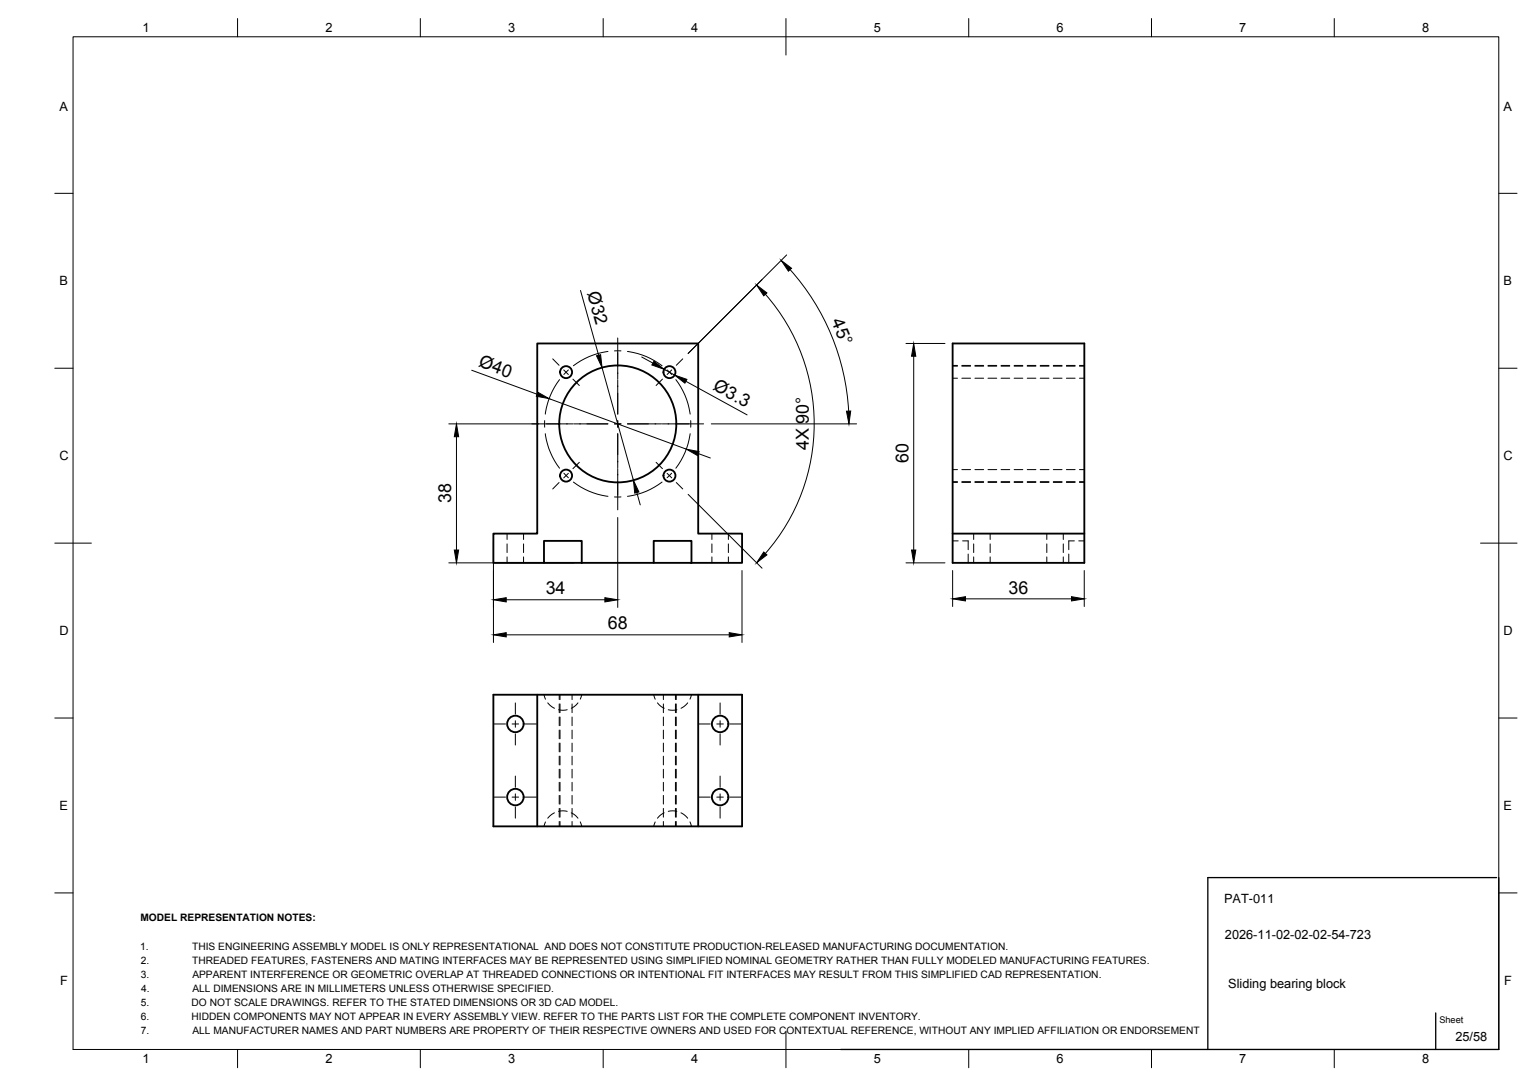
ISO-10303-21;
HEADER;
/* Generated by software containing ST-Developer
 * from STEP Tools, Inc. (www.steptools.com) 
 */

FILE_DESCRIPTION(
/* description */ ('Belt tension measurement rig'),
/* implementation_level */ '2;1');

FILE_NAME(
/* name */ 'Sliding bearing block.step',
/* time_stamp */ '2026-10-28T03:24:44-07:00',
/* author */ (''),
/* organization */ (''),
/* preprocessor_version */ 'ST-DEVELOPER v20.2',
/* originating_system */ 'Autodesk Translation Framework v15.17.0.0',
/* authorisation */ '');

FILE_SCHEMA (('AUTOMOTIVE_DESIGN { 1 0 10303 214 3 1 1 }'));
ENDSEC;

DATA;
#10=MECHANICAL_DESIGN_GEOMETRIC_PRESENTATION_REPRESENTATION('',(#720),#23587);
#602=SHAPE_REPRESENTATION_RELATIONSHIP('SRR','None',#23849,#657);
#657=ADVANCED_BREP_SHAPE_REPRESENTATION('',(#790),#23547);
#720=STYLED_ITEM('',(#24211),#790);
#790=MANIFOLD_SOLID_BREP('Body1',#12225);
#936=FACE_BOUND('',#2421,.T.);
#937=FACE_BOUND('',#2422,.T.);
#938=FACE_BOUND('',#2423,.T.);
#939=FACE_BOUND('',#2424,.T.);
#940=FACE_BOUND('',#2425,.T.);
#941=FACE_BOUND('',#2427,.T.);
#942=FACE_BOUND('',#2428,.T.);
#943=FACE_BOUND('',#2429,.T.);
#944=FACE_BOUND('',#2430,.T.);
#945=FACE_BOUND('',#2431,.T.);
#946=FACE_BOUND('',#2437,.T.);
#947=FACE_BOUND('',#2438,.T.);
#948=FACE_BOUND('',#2440,.T.);
#949=FACE_BOUND('',#2441,.T.);
#950=FACE_BOUND('',#2448,.T.);
#951=FACE_BOUND('',#2449,.T.);
#952=FACE_BOUND('',#2450,.T.);
#953=FACE_BOUND('',#2451,.T.);
#1161=PLANE('',#13409);
#1162=PLANE('',#13413);
#1163=PLANE('',#13417);
#1164=PLANE('',#13421);
#1165=PLANE('',#13425);
#1166=PLANE('',#13426);
#1167=PLANE('',#13439);
#1168=PLANE('',#13440);
#1169=PLANE('',#13441);
#1170=PLANE('',#13442);
#1171=PLANE('',#13443);
#1172=PLANE('',#13444);
#1173=PLANE('',#13445);
#1174=PLANE('',#13446);
#1596=FACE_OUTER_BOUND('',#2407,.T.);
#1597=FACE_OUTER_BOUND('',#2408,.T.);
#1598=FACE_OUTER_BOUND('',#2409,.T.);
#1599=FACE_OUTER_BOUND('',#2410,.T.);
#1600=FACE_OUTER_BOUND('',#2411,.T.);
#1601=FACE_OUTER_BOUND('',#2412,.T.);
#1602=FACE_OUTER_BOUND('',#2413,.T.);
#1603=FACE_OUTER_BOUND('',#2414,.T.);
#1604=FACE_OUTER_BOUND('',#2415,.T.);
#1605=FACE_OUTER_BOUND('',#2416,.T.);
#1606=FACE_OUTER_BOUND('',#2417,.T.);
#1607=FACE_OUTER_BOUND('',#2418,.T.);
#1608=FACE_OUTER_BOUND('',#2419,.T.);
#1609=FACE_OUTER_BOUND('',#2420,.T.);
#1610=FACE_OUTER_BOUND('',#2426,.T.);
#1611=FACE_OUTER_BOUND('',#2432,.T.);
#1612=FACE_OUTER_BOUND('',#2433,.T.);
#1613=FACE_OUTER_BOUND('',#2434,.T.);
#1614=FACE_OUTER_BOUND('',#2435,.T.);
#1615=FACE_OUTER_BOUND('',#2436,.T.);
#1616=FACE_OUTER_BOUND('',#2439,.T.);
#1617=FACE_OUTER_BOUND('',#2442,.T.);
#1618=FACE_OUTER_BOUND('',#2443,.T.);
#1619=FACE_OUTER_BOUND('',#2444,.T.);
#1620=FACE_OUTER_BOUND('',#2445,.T.);
#1621=FACE_OUTER_BOUND('',#2446,.T.);
#1622=FACE_OUTER_BOUND('',#2447,.T.);
#2407=EDGE_LOOP('',(#8980,#8981,#8982,#8983));
#2408=EDGE_LOOP('',(#8984,#8985,#8986,#8987));
#2409=EDGE_LOOP('',(#8988,#8989,#8990,#8991));
#2410=EDGE_LOOP('',(#8992,#8993,#8994,#8995));
#2411=EDGE_LOOP('',(#8996,#8997,#8998,#8999));
#2412=EDGE_LOOP('',(#9000,#9001));
#2413=EDGE_LOOP('',(#9002,#9003,#9004,#9005));
#2414=EDGE_LOOP('',(#9006,#9007));
#2415=EDGE_LOOP('',(#9008,#9009,#9010,#9011));
#2416=EDGE_LOOP('',(#9012,#9013));
#2417=EDGE_LOOP('',(#9014,#9015,#9016,#9017));
#2418=EDGE_LOOP('',(#9018,#9019));
#2419=EDGE_LOOP('',(#9020,#9021,#9022,#9023));
#2420=EDGE_LOOP('',(#9024,#9025,#9026,#9027,#9028,#9029,#9030,#9031,#9032,
#9033,#9034,#9035,#9036,#9037,#9038,#9039));
#2421=EDGE_LOOP('',(#9040));
#2422=EDGE_LOOP('',(#9041));
#2423=EDGE_LOOP('',(#9042));
#2424=EDGE_LOOP('',(#9043));
#2425=EDGE_LOOP('',(#9044));
#2426=EDGE_LOOP('',(#9045,#9046,#9047,#9048,#9049,#9050,#9051,#9052,#9053,
#9054,#9055,#9056,#9057,#9058,#9059,#9060));
#2427=EDGE_LOOP('',(#9061));
#2428=EDGE_LOOP('',(#9062));
#2429=EDGE_LOOP('',(#9063));
#2430=EDGE_LOOP('',(#9064));
#2431=EDGE_LOOP('',(#9065));
#2432=EDGE_LOOP('',(#9066,#9067,#9068,#9069));
#2433=EDGE_LOOP('',(#9070,#9071,#9072,#9073));
#2434=EDGE_LOOP('',(#9074,#9075,#9076,#9077));
#2435=EDGE_LOOP('',(#9078,#9079,#9080,#9081));
#2436=EDGE_LOOP('',(#9082,#9083,#9084,#9085));
#2437=EDGE_LOOP('',(#9086));
#2438=EDGE_LOOP('',(#9087));
#2439=EDGE_LOOP('',(#9088,#9089,#9090,#9091));
#2440=EDGE_LOOP('',(#9092));
#2441=EDGE_LOOP('',(#9093));
#2442=EDGE_LOOP('',(#9094,#9095,#9096,#9097));
#2443=EDGE_LOOP('',(#9098,#9099,#9100,#9101));
#2444=EDGE_LOOP('',(#9102,#9103,#9104,#9105));
#2445=EDGE_LOOP('',(#9106,#9107,#9108,#9109));
#2446=EDGE_LOOP('',(#9110,#9111,#9112,#9113));
#2447=EDGE_LOOP('',(#9114,#9115,#9116,#9117,#9118,#9119,#9120,#9121,#9122,
#9123,#9124,#9125));
#2448=EDGE_LOOP('',(#9126));
#2449=EDGE_LOOP('',(#9127));
#2450=EDGE_LOOP('',(#9128));
#2451=EDGE_LOOP('',(#9129));
#3223=LINE('',#20113,#3974);
#3224=LINE('',#20119,#3975);
#3225=LINE('',#20125,#3976);
#3226=LINE('',#20131,#3977);
#3227=LINE('',#20137,#3978);
#3228=LINE('',#20142,#3979);
#3229=LINE('',#20146,#3980);
#3230=LINE('',#20149,#3981);
#3231=LINE('',#20153,#3982);
#3232=LINE('',#20157,#3983);
#3233=LINE('',#20160,#3984);
#3234=LINE('',#20164,#3985);
#3235=LINE('',#20168,#3986);
#3236=LINE('',#20171,#3987);
#3237=LINE('',#20175,#3988);
#3238=LINE('',#20179,#3989);
#3239=LINE('',#20182,#3990);
#3240=LINE('',#20185,#3991);
#3241=LINE('',#20187,#3992);
#3242=LINE('',#20189,#3993);
#3243=LINE('',#20191,#3994);
#3244=LINE('',#20193,#3995);
#3245=LINE('',#20195,#3996);
#3246=LINE('',#20197,#3997);
#3247=LINE('',#20199,#3998);
#3248=LINE('',#20200,#3999);
#3249=LINE('',#20201,#4000);
#3250=LINE('',#20204,#4001);
#3251=LINE('',#20206,#4002);
#3252=LINE('',#20208,#4003);
#3253=LINE('',#20210,#4004);
#3254=LINE('',#20212,#4005);
#3255=LINE('',#20214,#4006);
#3256=LINE('',#20216,#4007);
#3257=LINE('',#20218,#4008);
#3258=LINE('',#20219,#4009);
#3259=LINE('',#20220,#4010);
#3260=LINE('',#20225,#4011);
#3261=LINE('',#20231,#4012);
#3262=LINE('',#20237,#4013);
#3263=LINE('',#20243,#4014);
#3264=LINE('',#20246,#4015);
#3265=LINE('',#20247,#4016);
#3266=LINE('',#20249,#4017);
#3267=LINE('',#20250,#4018);
#3268=LINE('',#20252,#4019);
#3269=LINE('',#20254,#4020);
#3270=LINE('',#20256,#4021);
#3271=LINE('',#20258,#4022);
#3974=VECTOR('',#15812,0.164999999999999);
#3975=VECTOR('',#15819,0.164999999999999);
#3976=VECTOR('',#15826,0.164999999999999);
#3977=VECTOR('',#15833,0.164999999999999);
#3978=VECTOR('',#15840,1.6);
#3979=VECTOR('',#15845,1.);
#3980=VECTOR('',#15850,1.);
#3981=VECTOR('',#15853,1.);
#3982=VECTOR('',#15856,1.);
#3983=VECTOR('',#15861,1.);
#3984=VECTOR('',#15864,1.);
#3985=VECTOR('',#15867,1.);
#3986=VECTOR('',#15872,1.);
#3987=VECTOR('',#15875,1.);
#3988=VECTOR('',#15878,1.);
#3989=VECTOR('',#15883,1.);
#3990=VECTOR('',#15886,1.);
#3991=VECTOR('',#15889,1.);
#3992=VECTOR('',#15890,1.);
#3993=VECTOR('',#15891,1.);
#3994=VECTOR('',#15892,1.);
#3995=VECTOR('',#15893,1.);
#3996=VECTOR('',#15894,1.);
#3997=VECTOR('',#15895,1.);
#3998=VECTOR('',#15896,1.);
#3999=VECTOR('',#15897,1.);
#4000=VECTOR('',#15898,1.);
#4001=VECTOR('',#15901,1.);
#4002=VECTOR('',#15902,1.);
#4003=VECTOR('',#15903,1.);
#4004=VECTOR('',#15904,1.);
#4005=VECTOR('',#15905,1.);
#4006=VECTOR('',#15906,1.);
#4007=VECTOR('',#15907,1.);
#4008=VECTOR('',#15908,1.);
#4009=VECTOR('',#15909,1.);
#4010=VECTOR('',#15910,1.);
#4011=VECTOR('',#15915,0.225);
#4012=VECTOR('',#15922,0.225);
#4013=VECTOR('',#15929,0.225);
#4014=VECTOR('',#15936,0.225);
#4015=VECTOR('',#15941,1.);
#4016=VECTOR('',#15942,1.);
#4017=VECTOR('',#15945,1.);
#4018=VECTOR('',#15946,1.);
#4019=VECTOR('',#15949,1.);
#4020=VECTOR('',#15952,1.);
#4021=VECTOR('',#15955,1.);
#4022=VECTOR('',#15958,1.);
#4714=CIRCLE('',#13395,0.164999999999999);
#4715=CIRCLE('',#13396,0.164999999999999);
#4716=CIRCLE('',#13398,0.164999999999999);
#4717=CIRCLE('',#13399,0.164999999999999);
#4718=CIRCLE('',#13401,0.164999999999999);
#4719=CIRCLE('',#13402,0.164999999999999);
#4720=CIRCLE('',#13404,0.164999999999999);
#4721=CIRCLE('',#13405,0.164999999999999);
#4722=CIRCLE('',#13407,1.6);
#4723=CIRCLE('',#13408,1.6);
#4724=CIRCLE('',#13410,0.525);
#4725=CIRCLE('',#13412,0.525);
#4726=CIRCLE('',#13414,0.525);
#4727=CIRCLE('',#13416,0.525);
#4728=CIRCLE('',#13418,0.525);
#4729=CIRCLE('',#13420,0.525);
#4730=CIRCLE('',#13422,0.525);
#4731=CIRCLE('',#13424,0.525);
#4732=CIRCLE('',#13428,0.225);
#4733=CIRCLE('',#13429,0.225);
#4734=CIRCLE('',#13431,0.225);
#4735=CIRCLE('',#13432,0.225);
#4736=CIRCLE('',#13434,0.225);
#4737=CIRCLE('',#13435,0.225);
#4738=CIRCLE('',#13437,0.225);
#4739=CIRCLE('',#13438,0.225);
#5592=VERTEX_POINT('',#20110);
#5593=VERTEX_POINT('',#20112);
#5594=VERTEX_POINT('',#20116);
#5595=VERTEX_POINT('',#20118);
#5596=VERTEX_POINT('',#20122);
#5597=VERTEX_POINT('',#20124);
#5598=VERTEX_POINT('',#20128);
#5599=VERTEX_POINT('',#20130);
#5600=VERTEX_POINT('',#20134);
#5601=VERTEX_POINT('',#20136);
#5602=VERTEX_POINT('',#20140);
#5603=VERTEX_POINT('',#20141);
#5604=VERTEX_POINT('',#20145);
#5605=VERTEX_POINT('',#20147);
#5606=VERTEX_POINT('',#20151);
#5607=VERTEX_POINT('',#20152);
#5608=VERTEX_POINT('',#20156);
#5609=VERTEX_POINT('',#20158);
#5610=VERTEX_POINT('',#20162);
#5611=VERTEX_POINT('',#20163);
#5612=VERTEX_POINT('',#20167);
#5613=VERTEX_POINT('',#20169);
#5614=VERTEX_POINT('',#20173);
#5615=VERTEX_POINT('',#20174);
#5616=VERTEX_POINT('',#20178);
#5617=VERTEX_POINT('',#20180);
#5618=VERTEX_POINT('',#20184);
#5619=VERTEX_POINT('',#20186);
#5620=VERTEX_POINT('',#20188);
#5621=VERTEX_POINT('',#20190);
#5622=VERTEX_POINT('',#20192);
#5623=VERTEX_POINT('',#20194);
#5624=VERTEX_POINT('',#20196);
#5625=VERTEX_POINT('',#20198);
#5626=VERTEX_POINT('',#20203);
#5627=VERTEX_POINT('',#20205);
#5628=VERTEX_POINT('',#20207);
#5629=VERTEX_POINT('',#20209);
#5630=VERTEX_POINT('',#20211);
#5631=VERTEX_POINT('',#20213);
#5632=VERTEX_POINT('',#20215);
#5633=VERTEX_POINT('',#20217);
#5634=VERTEX_POINT('',#20222);
#5635=VERTEX_POINT('',#20224);
#5636=VERTEX_POINT('',#20228);
#5637=VERTEX_POINT('',#20230);
#5638=VERTEX_POINT('',#20234);
#5639=VERTEX_POINT('',#20236);
#5640=VERTEX_POINT('',#20240);
#5641=VERTEX_POINT('',#20242);
#6849=EDGE_CURVE('',#5592,#5592,#4714,.T.);
#6850=EDGE_CURVE('',#5592,#5593,#3223,.T.);
#6851=EDGE_CURVE('',#5593,#5593,#4715,.T.);
#6852=EDGE_CURVE('',#5594,#5594,#4716,.T.);
#6853=EDGE_CURVE('',#5594,#5595,#3224,.T.);
#6854=EDGE_CURVE('',#5595,#5595,#4717,.T.);
#6855=EDGE_CURVE('',#5596,#5596,#4718,.T.);
#6856=EDGE_CURVE('',#5596,#5597,#3225,.T.);
#6857=EDGE_CURVE('',#5597,#5597,#4719,.T.);
#6858=EDGE_CURVE('',#5598,#5598,#4720,.T.);
#6859=EDGE_CURVE('',#5598,#5599,#3226,.T.);
#6860=EDGE_CURVE('',#5599,#5599,#4721,.T.);
#6861=EDGE_CURVE('',#5600,#5600,#4722,.T.);
#6862=EDGE_CURVE('',#5600,#5601,#3227,.T.);
#6863=EDGE_CURVE('',#5601,#5601,#4723,.T.);
#6864=EDGE_CURVE('',#5602,#5603,#3228,.T.);
#6865=EDGE_CURVE('',#5603,#5602,#4724,.T.);
#6866=EDGE_CURVE('',#5604,#5602,#3229,.T.);
#6867=EDGE_CURVE('',#5605,#5604,#4725,.T.);
#6868=EDGE_CURVE('',#5603,#5605,#3230,.T.);
#6869=EDGE_CURVE('',#5606,#5607,#3231,.T.);
#6870=EDGE_CURVE('',#5607,#5606,#4726,.T.);
#6871=EDGE_CURVE('',#5608,#5606,#3232,.T.);
#6872=EDGE_CURVE('',#5609,#5608,#4727,.T.);
#6873=EDGE_CURVE('',#5607,#5609,#3233,.T.);
#6874=EDGE_CURVE('',#5610,#5611,#3234,.T.);
#6875=EDGE_CURVE('',#5611,#5610,#4728,.T.);
#6876=EDGE_CURVE('',#5612,#5610,#3235,.T.);
#6877=EDGE_CURVE('',#5613,#5612,#4729,.T.);
#6878=EDGE_CURVE('',#5611,#5613,#3236,.T.);
#6879=EDGE_CURVE('',#5614,#5615,#3237,.T.);
#6880=EDGE_CURVE('',#5615,#5614,#4730,.T.);
#6881=EDGE_CURVE('',#5616,#5614,#3238,.T.);
#6882=EDGE_CURVE('',#5617,#5616,#4731,.T.);
#6883=EDGE_CURVE('',#5615,#5617,#3239,.T.);
#6884=EDGE_CURVE('',#5605,#5618,#3240,.T.);
#6885=EDGE_CURVE('',#5618,#5619,#3241,.T.);
#6886=EDGE_CURVE('',#5619,#5620,#3242,.T.);
#6887=EDGE_CURVE('',#5620,#5621,#3243,.T.);
#6888=EDGE_CURVE('',#5622,#5621,#3244,.T.);
#6889=EDGE_CURVE('',#5623,#5622,#3245,.T.);
#6890=EDGE_CURVE('',#5623,#5624,#3246,.T.);
#6891=EDGE_CURVE('',#5624,#5625,#3247,.T.);
#6892=EDGE_CURVE('',#5625,#5612,#3248,.T.);
#6893=EDGE_CURVE('',#5613,#5604,#3249,.T.);
#6894=EDGE_CURVE('',#5609,#5626,#3250,.T.);
#6895=EDGE_CURVE('',#5626,#5627,#3251,.T.);
#6896=EDGE_CURVE('',#5627,#5628,#3252,.T.);
#6897=EDGE_CURVE('',#5628,#5629,#3253,.T.);
#6898=EDGE_CURVE('',#5630,#5629,#3254,.T.);
#6899=EDGE_CURVE('',#5631,#5630,#3255,.T.);
#6900=EDGE_CURVE('',#5631,#5632,#3256,.T.);
#6901=EDGE_CURVE('',#5632,#5633,#3257,.T.);
#6902=EDGE_CURVE('',#5633,#5616,#3258,.T.);
#6903=EDGE_CURVE('',#5617,#5608,#3259,.T.);
#6904=EDGE_CURVE('',#5634,#5634,#4732,.T.);
#6905=EDGE_CURVE('',#5634,#5635,#3260,.T.);
#6906=EDGE_CURVE('',#5635,#5635,#4733,.T.);
#6907=EDGE_CURVE('',#5636,#5636,#4734,.T.);
#6908=EDGE_CURVE('',#5636,#5637,#3261,.T.);
#6909=EDGE_CURVE('',#5637,#5637,#4735,.T.);
#6910=EDGE_CURVE('',#5638,#5638,#4736,.T.);
#6911=EDGE_CURVE('',#5638,#5639,#3262,.T.);
#6912=EDGE_CURVE('',#5639,#5639,#4737,.T.);
#6913=EDGE_CURVE('',#5640,#5640,#4738,.T.);
#6914=EDGE_CURVE('',#5640,#5641,#3263,.T.);
#6915=EDGE_CURVE('',#5641,#5641,#4739,.T.);
#6916=EDGE_CURVE('',#5620,#5631,#3264,.T.);
#6917=EDGE_CURVE('',#5619,#5632,#3265,.T.);
#6918=EDGE_CURVE('',#5628,#5623,#3266,.T.);
#6919=EDGE_CURVE('',#5624,#5627,#3267,.T.);
#6920=EDGE_CURVE('',#5625,#5626,#3268,.T.);
#6921=EDGE_CURVE('',#5618,#5633,#3269,.T.);
#6922=EDGE_CURVE('',#5621,#5630,#3270,.T.);
#6923=EDGE_CURVE('',#5629,#5622,#3271,.T.);
#8980=ORIENTED_EDGE('',*,*,#6849,.F.);
#8981=ORIENTED_EDGE('',*,*,#6850,.T.);
#8982=ORIENTED_EDGE('',*,*,#6851,.F.);
#8983=ORIENTED_EDGE('',*,*,#6850,.F.);
#8984=ORIENTED_EDGE('',*,*,#6852,.F.);
#8985=ORIENTED_EDGE('',*,*,#6853,.T.);
#8986=ORIENTED_EDGE('',*,*,#6854,.F.);
#8987=ORIENTED_EDGE('',*,*,#6853,.F.);
#8988=ORIENTED_EDGE('',*,*,#6855,.F.);
#8989=ORIENTED_EDGE('',*,*,#6856,.T.);
#8990=ORIENTED_EDGE('',*,*,#6857,.F.);
#8991=ORIENTED_EDGE('',*,*,#6856,.F.);
#8992=ORIENTED_EDGE('',*,*,#6858,.F.);
#8993=ORIENTED_EDGE('',*,*,#6859,.T.);
#8994=ORIENTED_EDGE('',*,*,#6860,.F.);
#8995=ORIENTED_EDGE('',*,*,#6859,.F.);
#8996=ORIENTED_EDGE('',*,*,#6861,.F.);
#8997=ORIENTED_EDGE('',*,*,#6862,.T.);
#8998=ORIENTED_EDGE('',*,*,#6863,.F.);
#8999=ORIENTED_EDGE('',*,*,#6862,.F.);
#9000=ORIENTED_EDGE('',*,*,#6864,.F.);
#9001=ORIENTED_EDGE('',*,*,#6865,.F.);
#9002=ORIENTED_EDGE('',*,*,#6866,.F.);
#9003=ORIENTED_EDGE('',*,*,#6867,.F.);
#9004=ORIENTED_EDGE('',*,*,#6868,.F.);
#9005=ORIENTED_EDGE('',*,*,#6865,.T.);
#9006=ORIENTED_EDGE('',*,*,#6869,.F.);
#9007=ORIENTED_EDGE('',*,*,#6870,.F.);
#9008=ORIENTED_EDGE('',*,*,#6871,.F.);
#9009=ORIENTED_EDGE('',*,*,#6872,.F.);
#9010=ORIENTED_EDGE('',*,*,#6873,.F.);
#9011=ORIENTED_EDGE('',*,*,#6870,.T.);
#9012=ORIENTED_EDGE('',*,*,#6874,.F.);
#9013=ORIENTED_EDGE('',*,*,#6875,.F.);
#9014=ORIENTED_EDGE('',*,*,#6876,.F.);
#9015=ORIENTED_EDGE('',*,*,#6877,.F.);
#9016=ORIENTED_EDGE('',*,*,#6878,.F.);
#9017=ORIENTED_EDGE('',*,*,#6875,.T.);
#9018=ORIENTED_EDGE('',*,*,#6879,.F.);
#9019=ORIENTED_EDGE('',*,*,#6880,.F.);
#9020=ORIENTED_EDGE('',*,*,#6881,.F.);
#9021=ORIENTED_EDGE('',*,*,#6882,.F.);
#9022=ORIENTED_EDGE('',*,*,#6883,.F.);
#9023=ORIENTED_EDGE('',*,*,#6880,.T.);
#9024=ORIENTED_EDGE('',*,*,#6866,.T.);
#9025=ORIENTED_EDGE('',*,*,#6864,.T.);
#9026=ORIENTED_EDGE('',*,*,#6868,.T.);
#9027=ORIENTED_EDGE('',*,*,#6884,.T.);
#9028=ORIENTED_EDGE('',*,*,#6885,.T.);
#9029=ORIENTED_EDGE('',*,*,#6886,.T.);
#9030=ORIENTED_EDGE('',*,*,#6887,.T.);
#9031=ORIENTED_EDGE('',*,*,#6888,.F.);
#9032=ORIENTED_EDGE('',*,*,#6889,.F.);
#9033=ORIENTED_EDGE('',*,*,#6890,.T.);
#9034=ORIENTED_EDGE('',*,*,#6891,.T.);
#9035=ORIENTED_EDGE('',*,*,#6892,.T.);
#9036=ORIENTED_EDGE('',*,*,#6876,.T.);
#9037=ORIENTED_EDGE('',*,*,#6874,.T.);
#9038=ORIENTED_EDGE('',*,*,#6878,.T.);
#9039=ORIENTED_EDGE('',*,*,#6893,.T.);
#9040=ORIENTED_EDGE('',*,*,#6861,.T.);
#9041=ORIENTED_EDGE('',*,*,#6858,.T.);
#9042=ORIENTED_EDGE('',*,*,#6855,.T.);
#9043=ORIENTED_EDGE('',*,*,#6852,.T.);
#9044=ORIENTED_EDGE('',*,*,#6849,.T.);
#9045=ORIENTED_EDGE('',*,*,#6871,.T.);
#9046=ORIENTED_EDGE('',*,*,#6869,.T.);
#9047=ORIENTED_EDGE('',*,*,#6873,.T.);
#9048=ORIENTED_EDGE('',*,*,#6894,.T.);
#9049=ORIENTED_EDGE('',*,*,#6895,.T.);
#9050=ORIENTED_EDGE('',*,*,#6896,.T.);
#9051=ORIENTED_EDGE('',*,*,#6897,.T.);
#9052=ORIENTED_EDGE('',*,*,#6898,.F.);
#9053=ORIENTED_EDGE('',*,*,#6899,.F.);
#9054=ORIENTED_EDGE('',*,*,#6900,.T.);
#9055=ORIENTED_EDGE('',*,*,#6901,.T.);
#9056=ORIENTED_EDGE('',*,*,#6902,.T.);
#9057=ORIENTED_EDGE('',*,*,#6881,.T.);
#9058=ORIENTED_EDGE('',*,*,#6879,.T.);
#9059=ORIENTED_EDGE('',*,*,#6883,.T.);
#9060=ORIENTED_EDGE('',*,*,#6903,.T.);
#9061=ORIENTED_EDGE('',*,*,#6863,.T.);
#9062=ORIENTED_EDGE('',*,*,#6860,.T.);
#9063=ORIENTED_EDGE('',*,*,#6857,.T.);
#9064=ORIENTED_EDGE('',*,*,#6854,.T.);
#9065=ORIENTED_EDGE('',*,*,#6851,.T.);
#9066=ORIENTED_EDGE('',*,*,#6904,.F.);
#9067=ORIENTED_EDGE('',*,*,#6905,.T.);
#9068=ORIENTED_EDGE('',*,*,#6906,.F.);
#9069=ORIENTED_EDGE('',*,*,#6905,.F.);
#9070=ORIENTED_EDGE('',*,*,#6907,.F.);
#9071=ORIENTED_EDGE('',*,*,#6908,.T.);
#9072=ORIENTED_EDGE('',*,*,#6909,.F.);
#9073=ORIENTED_EDGE('',*,*,#6908,.F.);
#9074=ORIENTED_EDGE('',*,*,#6910,.F.);
#9075=ORIENTED_EDGE('',*,*,#6911,.T.);
#9076=ORIENTED_EDGE('',*,*,#6912,.F.);
#9077=ORIENTED_EDGE('',*,*,#6911,.F.);
#9078=ORIENTED_EDGE('',*,*,#6913,.F.);
#9079=ORIENTED_EDGE('',*,*,#6914,.T.);
#9080=ORIENTED_EDGE('',*,*,#6915,.F.);
#9081=ORIENTED_EDGE('',*,*,#6914,.F.);
#9082=ORIENTED_EDGE('',*,*,#6916,.F.);
#9083=ORIENTED_EDGE('',*,*,#6886,.F.);
#9084=ORIENTED_EDGE('',*,*,#6917,.T.);
#9085=ORIENTED_EDGE('',*,*,#6900,.F.);
#9086=ORIENTED_EDGE('',*,*,#6906,.T.);
#9087=ORIENTED_EDGE('',*,*,#6915,.T.);
#9088=ORIENTED_EDGE('',*,*,#6918,.F.);
#9089=ORIENTED_EDGE('',*,*,#6896,.F.);
#9090=ORIENTED_EDGE('',*,*,#6919,.F.);
#9091=ORIENTED_EDGE('',*,*,#6890,.F.);
#9092=ORIENTED_EDGE('',*,*,#6909,.T.);
#9093=ORIENTED_EDGE('',*,*,#6912,.T.);
#9094=ORIENTED_EDGE('',*,*,#6891,.F.);
#9095=ORIENTED_EDGE('',*,*,#6919,.T.);
#9096=ORIENTED_EDGE('',*,*,#6895,.F.);
#9097=ORIENTED_EDGE('',*,*,#6920,.F.);
#9098=ORIENTED_EDGE('',*,*,#6885,.F.);
#9099=ORIENTED_EDGE('',*,*,#6921,.T.);
#9100=ORIENTED_EDGE('',*,*,#6901,.F.);
#9101=ORIENTED_EDGE('',*,*,#6917,.F.);
#9102=ORIENTED_EDGE('',*,*,#6916,.T.);
#9103=ORIENTED_EDGE('',*,*,#6899,.T.);
#9104=ORIENTED_EDGE('',*,*,#6922,.F.);
#9105=ORIENTED_EDGE('',*,*,#6887,.F.);
#9106=ORIENTED_EDGE('',*,*,#6918,.T.);
#9107=ORIENTED_EDGE('',*,*,#6889,.T.);
#9108=ORIENTED_EDGE('',*,*,#6923,.F.);
#9109=ORIENTED_EDGE('',*,*,#6897,.F.);
#9110=ORIENTED_EDGE('',*,*,#6923,.T.);
#9111=ORIENTED_EDGE('',*,*,#6888,.T.);
#9112=ORIENTED_EDGE('',*,*,#6922,.T.);
#9113=ORIENTED_EDGE('',*,*,#6898,.T.);
#9114=ORIENTED_EDGE('',*,*,#6867,.T.);
#9115=ORIENTED_EDGE('',*,*,#6893,.F.);
#9116=ORIENTED_EDGE('',*,*,#6877,.T.);
#9117=ORIENTED_EDGE('',*,*,#6892,.F.);
#9118=ORIENTED_EDGE('',*,*,#6920,.T.);
#9119=ORIENTED_EDGE('',*,*,#6894,.F.);
#9120=ORIENTED_EDGE('',*,*,#6872,.T.);
#9121=ORIENTED_EDGE('',*,*,#6903,.F.);
#9122=ORIENTED_EDGE('',*,*,#6882,.T.);
#9123=ORIENTED_EDGE('',*,*,#6902,.F.);
#9124=ORIENTED_EDGE('',*,*,#6921,.F.);
#9125=ORIENTED_EDGE('',*,*,#6884,.F.);
#9126=ORIENTED_EDGE('',*,*,#6904,.T.);
#9127=ORIENTED_EDGE('',*,*,#6907,.T.);
#9128=ORIENTED_EDGE('',*,*,#6910,.T.);
#9129=ORIENTED_EDGE('',*,*,#6913,.T.);
#11256=CYLINDRICAL_SURFACE('',#13394,0.164999999999999);
#11257=CYLINDRICAL_SURFACE('',#13397,0.164999999999999);
#11258=CYLINDRICAL_SURFACE('',#13400,0.164999999999999);
#11259=CYLINDRICAL_SURFACE('',#13403,0.164999999999999);
#11260=CYLINDRICAL_SURFACE('',#13406,1.6);
#11261=CYLINDRICAL_SURFACE('',#13411,0.525);
#11262=CYLINDRICAL_SURFACE('',#13415,0.525);
#11263=CYLINDRICAL_SURFACE('',#13419,0.525);
#11264=CYLINDRICAL_SURFACE('',#13423,0.525);
#11265=CYLINDRICAL_SURFACE('',#13427,0.225);
#11266=CYLINDRICAL_SURFACE('',#13430,0.225);
#11267=CYLINDRICAL_SURFACE('',#13433,0.225);
#11268=CYLINDRICAL_SURFACE('',#13436,0.225);
#11737=ADVANCED_FACE('',(#1596),#11256,.F.);
#11738=ADVANCED_FACE('',(#1597),#11257,.F.);
#11739=ADVANCED_FACE('',(#1598),#11258,.F.);
#11740=ADVANCED_FACE('',(#1599),#11259,.F.);
#11741=ADVANCED_FACE('',(#1600),#11260,.F.);
#11742=ADVANCED_FACE('',(#1601),#1161,.F.);
#11743=ADVANCED_FACE('',(#1602),#11261,.F.);
#11744=ADVANCED_FACE('',(#1603),#1162,.F.);
#11745=ADVANCED_FACE('',(#1604),#11262,.F.);
#11746=ADVANCED_FACE('',(#1605),#1163,.F.);
#11747=ADVANCED_FACE('',(#1606),#11263,.F.);
#11748=ADVANCED_FACE('',(#1607),#1164,.F.);
#11749=ADVANCED_FACE('',(#1608),#11264,.F.);
#11750=ADVANCED_FACE('',(#1609,#936,#937,#938,#939,#940),#1165,.T.);
#11751=ADVANCED_FACE('',(#1610,#941,#942,#943,#944,#945),#1166,.T.);
#11752=ADVANCED_FACE('',(#1611),#11265,.F.);
#11753=ADVANCED_FACE('',(#1612),#11266,.F.);
#11754=ADVANCED_FACE('',(#1613),#11267,.F.);
#11755=ADVANCED_FACE('',(#1614),#11268,.F.);
#11756=ADVANCED_FACE('',(#1615,#946,#947),#1167,.T.);
#11757=ADVANCED_FACE('',(#1616,#948,#949),#1168,.T.);
#11758=ADVANCED_FACE('',(#1617),#1169,.T.);
#11759=ADVANCED_FACE('',(#1618),#1170,.T.);
#11760=ADVANCED_FACE('',(#1619),#1171,.T.);
#11761=ADVANCED_FACE('',(#1620),#1172,.T.);
#11762=ADVANCED_FACE('',(#1621),#1173,.T.);
#11763=ADVANCED_FACE('',(#1622,#950,#951,#952,#953),#1174,.F.);
#12225=CLOSED_SHELL('',(#11737,#11738,#11739,#11740,#11741,#11742,#11743,
#11744,#11745,#11746,#11747,#11748,#11749,#11750,#11751,#11752,#11753,#11754,
#11755,#11756,#11757,#11758,#11759,#11760,#11761,#11762,#11763));
#13393=AXIS2_PLACEMENT_3D('',#20108,#15806,#15807);
#13394=AXIS2_PLACEMENT_3D('',#20109,#15808,#15809);
#13395=AXIS2_PLACEMENT_3D('',#20111,#15810,#15811);
#13396=AXIS2_PLACEMENT_3D('',#20114,#15813,#15814);
#13397=AXIS2_PLACEMENT_3D('',#20115,#15815,#15816);
#13398=AXIS2_PLACEMENT_3D('',#20117,#15817,#15818);
#13399=AXIS2_PLACEMENT_3D('',#20120,#15820,#15821);
#13400=AXIS2_PLACEMENT_3D('',#20121,#15822,#15823);
#13401=AXIS2_PLACEMENT_3D('',#20123,#15824,#15825);
#13402=AXIS2_PLACEMENT_3D('',#20126,#15827,#15828);
#13403=AXIS2_PLACEMENT_3D('',#20127,#15829,#15830);
#13404=AXIS2_PLACEMENT_3D('',#20129,#15831,#15832);
#13405=AXIS2_PLACEMENT_3D('',#20132,#15834,#15835);
#13406=AXIS2_PLACEMENT_3D('',#20133,#15836,#15837);
#13407=AXIS2_PLACEMENT_3D('',#20135,#15838,#15839);
#13408=AXIS2_PLACEMENT_3D('',#20138,#15841,#15842);
#13409=AXIS2_PLACEMENT_3D('',#20139,#15843,#15844);
#13410=AXIS2_PLACEMENT_3D('',#20143,#15846,#15847);
#13411=AXIS2_PLACEMENT_3D('',#20144,#15848,#15849);
#13412=AXIS2_PLACEMENT_3D('',#20148,#15851,#15852);
#13413=AXIS2_PLACEMENT_3D('',#20150,#15854,#15855);
#13414=AXIS2_PLACEMENT_3D('',#20154,#15857,#15858);
#13415=AXIS2_PLACEMENT_3D('',#20155,#15859,#15860);
#13416=AXIS2_PLACEMENT_3D('',#20159,#15862,#15863);
#13417=AXIS2_PLACEMENT_3D('',#20161,#15865,#15866);
#13418=AXIS2_PLACEMENT_3D('',#20165,#15868,#15869);
#13419=AXIS2_PLACEMENT_3D('',#20166,#15870,#15871);
#13420=AXIS2_PLACEMENT_3D('',#20170,#15873,#15874);
#13421=AXIS2_PLACEMENT_3D('',#20172,#15876,#15877);
#13422=AXIS2_PLACEMENT_3D('',#20176,#15879,#15880);
#13423=AXIS2_PLACEMENT_3D('',#20177,#15881,#15882);
#13424=AXIS2_PLACEMENT_3D('',#20181,#15884,#15885);
#13425=AXIS2_PLACEMENT_3D('',#20183,#15887,#15888);
#13426=AXIS2_PLACEMENT_3D('',#20202,#15899,#15900);
#13427=AXIS2_PLACEMENT_3D('',#20221,#15911,#15912);
#13428=AXIS2_PLACEMENT_3D('',#20223,#15913,#15914);
#13429=AXIS2_PLACEMENT_3D('',#20226,#15916,#15917);
#13430=AXIS2_PLACEMENT_3D('',#20227,#15918,#15919);
#13431=AXIS2_PLACEMENT_3D('',#20229,#15920,#15921);
#13432=AXIS2_PLACEMENT_3D('',#20232,#15923,#15924);
#13433=AXIS2_PLACEMENT_3D('',#20233,#15925,#15926);
#13434=AXIS2_PLACEMENT_3D('',#20235,#15927,#15928);
#13435=AXIS2_PLACEMENT_3D('',#20238,#15930,#15931);
#13436=AXIS2_PLACEMENT_3D('',#20239,#15932,#15933);
#13437=AXIS2_PLACEMENT_3D('',#20241,#15934,#15935);
#13438=AXIS2_PLACEMENT_3D('',#20244,#15937,#15938);
#13439=AXIS2_PLACEMENT_3D('',#20245,#15939,#15940);
#13440=AXIS2_PLACEMENT_3D('',#20248,#15943,#15944);
#13441=AXIS2_PLACEMENT_3D('',#20251,#15947,#15948);
#13442=AXIS2_PLACEMENT_3D('',#20253,#15950,#15951);
#13443=AXIS2_PLACEMENT_3D('',#20255,#15953,#15954);
#13444=AXIS2_PLACEMENT_3D('',#20257,#15956,#15957);
#13445=AXIS2_PLACEMENT_3D('',#20259,#15959,#15960);
#13446=AXIS2_PLACEMENT_3D('',#20260,#15961,#15962);
#15806=DIRECTION('axis',(0.,0.,1.));
#15807=DIRECTION('refdir',(1.,0.,0.));
#15808=DIRECTION('center_axis',(0.,1.,0.));
#15809=DIRECTION('ref_axis',(1.,0.,0.));
#15810=DIRECTION('center_axis',(0.,1.,0.));
#15811=DIRECTION('ref_axis',(1.,0.,0.));
#15812=DIRECTION('',(0.,1.,0.));
#15813=DIRECTION('center_axis',(0.,-1.,0.));
#15814=DIRECTION('ref_axis',(1.,0.,0.));
#15815=DIRECTION('center_axis',(0.,1.,0.));
#15816=DIRECTION('ref_axis',(1.,0.,0.));
#15817=DIRECTION('center_axis',(0.,1.,0.));
#15818=DIRECTION('ref_axis',(1.,0.,0.));
#15819=DIRECTION('',(0.,1.,0.));
#15820=DIRECTION('center_axis',(0.,-1.,0.));
#15821=DIRECTION('ref_axis',(1.,0.,0.));
#15822=DIRECTION('center_axis',(0.,1.,0.));
#15823=DIRECTION('ref_axis',(1.,0.,0.));
#15824=DIRECTION('center_axis',(0.,1.,0.));
#15825=DIRECTION('ref_axis',(1.,0.,0.));
#15826=DIRECTION('',(0.,1.,0.));
#15827=DIRECTION('center_axis',(0.,-1.,0.));
#15828=DIRECTION('ref_axis',(1.,0.,0.));
#15829=DIRECTION('center_axis',(0.,1.,0.));
#15830=DIRECTION('ref_axis',(1.,0.,0.));
#15831=DIRECTION('center_axis',(0.,1.,0.));
#15832=DIRECTION('ref_axis',(1.,0.,0.));
#15833=DIRECTION('',(0.,1.,0.));
#15834=DIRECTION('center_axis',(0.,-1.,0.));
#15835=DIRECTION('ref_axis',(1.,0.,0.));
#15836=DIRECTION('center_axis',(0.,1.,0.));
#15837=DIRECTION('ref_axis',(1.,0.,0.));
#15838=DIRECTION('center_axis',(0.,1.,0.));
#15839=DIRECTION('ref_axis',(1.,0.,0.));
#15840=DIRECTION('',(0.,1.,0.));
#15841=DIRECTION('center_axis',(0.,-1.,0.));
#15842=DIRECTION('ref_axis',(1.,0.,0.));
#15843=DIRECTION('center_axis',(0.,0.,1.));
#15844=DIRECTION('ref_axis',(1.,0.,0.));
#15845=DIRECTION('',(1.,0.,0.));
#15846=DIRECTION('center_axis',(0.,0.,1.));
#15847=DIRECTION('ref_axis',(1.,0.,0.));
#15848=DIRECTION('center_axis',(0.,0.,1.));
#15849=DIRECTION('ref_axis',(1.,0.,0.));
#15850=DIRECTION('',(0.,0.,1.));
#15851=DIRECTION('center_axis',(0.,0.,1.));
#15852=DIRECTION('ref_axis',(1.,0.,0.));
#15853=DIRECTION('',(0.,0.,-1.));
#15854=DIRECTION('center_axis',(0.,0.,1.));
#15855=DIRECTION('ref_axis',(1.,0.,0.));
#15856=DIRECTION('',(-1.,0.,0.));
#15857=DIRECTION('center_axis',(0.,0.,1.));
#15858=DIRECTION('ref_axis',(1.,0.,0.));
#15859=DIRECTION('center_axis',(0.,0.,1.));
#15860=DIRECTION('ref_axis',(1.,0.,0.));
#15861=DIRECTION('',(0.,0.,1.));
#15862=DIRECTION('center_axis',(0.,0.,1.));
#15863=DIRECTION('ref_axis',(1.,0.,0.));
#15864=DIRECTION('',(0.,0.,-1.));
#15865=DIRECTION('center_axis',(0.,0.,1.));
#15866=DIRECTION('ref_axis',(1.,0.,0.));
#15867=DIRECTION('',(1.,0.,0.));
#15868=DIRECTION('center_axis',(0.,0.,1.));
#15869=DIRECTION('ref_axis',(1.,0.,0.));
#15870=DIRECTION('center_axis',(0.,0.,1.));
#15871=DIRECTION('ref_axis',(1.,0.,0.));
#15872=DIRECTION('',(0.,0.,1.));
#15873=DIRECTION('center_axis',(0.,0.,1.));
#15874=DIRECTION('ref_axis',(1.,0.,0.));
#15875=DIRECTION('',(0.,0.,-1.));
#15876=DIRECTION('center_axis',(0.,0.,1.));
#15877=DIRECTION('ref_axis',(1.,0.,0.));
#15878=DIRECTION('',(-1.,0.,0.));
#15879=DIRECTION('center_axis',(0.,0.,1.));
#15880=DIRECTION('ref_axis',(1.,0.,0.));
#15881=DIRECTION('center_axis',(0.,0.,1.));
#15882=DIRECTION('ref_axis',(1.,0.,0.));
#15883=DIRECTION('',(0.,0.,1.));
#15884=DIRECTION('center_axis',(0.,0.,1.));
#15885=DIRECTION('ref_axis',(1.,0.,0.));
#15886=DIRECTION('',(0.,0.,-1.));
#15887=DIRECTION('center_axis',(0.,-1.,0.));
#15888=DIRECTION('ref_axis',(1.,0.,0.));
#15889=DIRECTION('',(1.,0.,0.));
#15890=DIRECTION('',(0.,0.,1.));
#15891=DIRECTION('',(-1.,0.,0.));
#15892=DIRECTION('',(0.,0.,1.));
#15893=DIRECTION('',(1.,0.,0.));
#15894=DIRECTION('',(0.,0.,1.));
#15895=DIRECTION('',(-1.,0.,0.));
#15896=DIRECTION('',(0.,0.,-1.));
#15897=DIRECTION('',(1.,0.,0.));
#15898=DIRECTION('',(1.,0.,0.));
#15899=DIRECTION('center_axis',(0.,1.,0.));
#15900=DIRECTION('ref_axis',(-1.,0.,0.));
#15901=DIRECTION('',(-1.,0.,0.));
#15902=DIRECTION('',(0.,0.,1.));
#15903=DIRECTION('',(1.,0.,0.));
#15904=DIRECTION('',(0.,0.,1.));
#15905=DIRECTION('',(-1.,0.,0.));
#15906=DIRECTION('',(0.,0.,1.));
#15907=DIRECTION('',(1.,0.,0.));
#15908=DIRECTION('',(0.,0.,-1.));
#15909=DIRECTION('',(-1.,0.,0.));
#15910=DIRECTION('',(-1.,0.,0.));
#15911=DIRECTION('center_axis',(0.,0.,1.));
#15912=DIRECTION('ref_axis',(1.,0.,0.));
#15913=DIRECTION('center_axis',(0.,0.,1.));
#15914=DIRECTION('ref_axis',(1.,0.,0.));
#15915=DIRECTION('',(0.,0.,1.));
#15916=DIRECTION('center_axis',(0.,0.,-1.));
#15917=DIRECTION('ref_axis',(1.,0.,0.));
#15918=DIRECTION('center_axis',(0.,0.,1.));
#15919=DIRECTION('ref_axis',(1.,0.,0.));
#15920=DIRECTION('center_axis',(0.,0.,1.));
#15921=DIRECTION('ref_axis',(1.,0.,0.));
#15922=DIRECTION('',(0.,0.,1.));
#15923=DIRECTION('center_axis',(0.,0.,-1.));
#15924=DIRECTION('ref_axis',(1.,0.,0.));
#15925=DIRECTION('center_axis',(0.,0.,1.));
#15926=DIRECTION('ref_axis',(1.,0.,0.));
#15927=DIRECTION('center_axis',(0.,0.,1.));
#15928=DIRECTION('ref_axis',(1.,0.,0.));
#15929=DIRECTION('',(0.,0.,1.));
#15930=DIRECTION('center_axis',(0.,0.,-1.));
#15931=DIRECTION('ref_axis',(1.,0.,0.));
#15932=DIRECTION('center_axis',(0.,0.,1.));
#15933=DIRECTION('ref_axis',(1.,0.,0.));
#15934=DIRECTION('center_axis',(0.,0.,1.));
#15935=DIRECTION('ref_axis',(1.,0.,0.));
#15936=DIRECTION('',(0.,0.,1.));
#15937=DIRECTION('center_axis',(0.,0.,-1.));
#15938=DIRECTION('ref_axis',(1.,0.,0.));
#15939=DIRECTION('center_axis',(0.,0.,1.));
#15940=DIRECTION('ref_axis',(1.,0.,0.));
#15941=DIRECTION('',(0.,1.,0.));
#15942=DIRECTION('',(0.,1.,0.));
#15943=DIRECTION('center_axis',(0.,0.,1.));
#15944=DIRECTION('ref_axis',(1.,0.,0.));
#15945=DIRECTION('',(0.,-1.,0.));
#15946=DIRECTION('',(0.,1.,0.));
#15947=DIRECTION('center_axis',(-1.,0.,0.));
#15948=DIRECTION('ref_axis',(0.,0.,1.));
#15949=DIRECTION('',(0.,1.,0.));
#15950=DIRECTION('center_axis',(1.,0.,0.));
#15951=DIRECTION('ref_axis',(0.,0.,-1.));
#15952=DIRECTION('',(0.,1.,0.));
#15953=DIRECTION('center_axis',(1.,0.,0.));
#15954=DIRECTION('ref_axis',(0.,1.,0.));
#15955=DIRECTION('',(0.,1.,0.));
#15956=DIRECTION('center_axis',(-1.,0.,0.));
#15957=DIRECTION('ref_axis',(0.,-1.,0.));
#15958=DIRECTION('',(0.,-1.,0.));
#15959=DIRECTION('center_axis',(0.,0.,1.));
#15960=DIRECTION('ref_axis',(1.,0.,0.));
#15961=DIRECTION('center_axis',(0.,0.,1.));
#15962=DIRECTION('ref_axis',(1.,0.,0.));
#20108=CARTESIAN_POINT('',(0.,0.,0.));
#20109=CARTESIAN_POINT('Origin',(8.5857864376269,-1.9,5.58578643762691));
#20110=CARTESIAN_POINT('',(8.42078643762691,-1.8,5.58578643762691));
#20111=CARTESIAN_POINT('Origin',(8.5857864376269,-1.8,5.58578643762691));
#20112=CARTESIAN_POINT('',(8.42078643762691,1.8,5.58578643762691));
#20113=CARTESIAN_POINT('',(8.42078643762691,-1.9,5.58578643762691));
#20114=CARTESIAN_POINT('Origin',(8.5857864376269,1.8,5.58578643762691));
#20115=CARTESIAN_POINT('Origin',(8.5857864376269,-1.9,8.4142135623731));
#20116=CARTESIAN_POINT('',(8.42078643762691,-1.8,8.4142135623731));
#20117=CARTESIAN_POINT('Origin',(8.5857864376269,-1.8,8.4142135623731));
#20118=CARTESIAN_POINT('',(8.42078643762691,1.8,8.4142135623731));
#20119=CARTESIAN_POINT('',(8.42078643762691,-1.9,8.4142135623731));
#20120=CARTESIAN_POINT('Origin',(8.5857864376269,1.8,8.4142135623731));
#20121=CARTESIAN_POINT('Origin',(11.4142135623731,-1.9,8.4142135623731));
#20122=CARTESIAN_POINT('',(11.2492135623731,-1.8,8.4142135623731));
#20123=CARTESIAN_POINT('Origin',(11.4142135623731,-1.8,8.4142135623731));
#20124=CARTESIAN_POINT('',(11.2492135623731,1.8,8.4142135623731));
#20125=CARTESIAN_POINT('',(11.2492135623731,-1.9,8.4142135623731));
#20126=CARTESIAN_POINT('Origin',(11.4142135623731,1.8,8.4142135623731));
#20127=CARTESIAN_POINT('Origin',(11.4142135623731,-1.9,5.58578643762691));
#20128=CARTESIAN_POINT('',(11.2492135623731,-1.8,5.58578643762691));
#20129=CARTESIAN_POINT('Origin',(11.4142135623731,-1.8,5.58578643762691));
#20130=CARTESIAN_POINT('',(11.2492135623731,1.8,5.58578643762691));
#20131=CARTESIAN_POINT('',(11.2492135623731,-1.9,5.58578643762691));
#20132=CARTESIAN_POINT('Origin',(11.4142135623731,1.8,5.58578643762691));
#20133=CARTESIAN_POINT('Origin',(10.,-1.9,7.));
#20134=CARTESIAN_POINT('',(8.4,-1.8,7.));
#20135=CARTESIAN_POINT('Origin',(10.,-1.8,7.));
#20136=CARTESIAN_POINT('',(8.4,1.8,7.));
#20137=CARTESIAN_POINT('',(8.4,-1.9,7.));
#20138=CARTESIAN_POINT('Origin',(10.,1.8,7.));
#20139=CARTESIAN_POINT('Origin',(11.5,-1.9,3.8));
#20140=CARTESIAN_POINT('',(10.9846117967978,-1.8,3.8));
#20141=CARTESIAN_POINT('',(12.0153882032022,-1.8,3.8));
#20142=CARTESIAN_POINT('',(9.65,-1.8,3.8));
#20143=CARTESIAN_POINT('Origin',(11.5,-1.9,3.8));
#20144=CARTESIAN_POINT('Origin',(11.5,-1.9,3.1));
#20145=CARTESIAN_POINT('',(10.9846117967978,-1.8,3.2));
#20146=CARTESIAN_POINT('',(10.9846117967978,-1.8,3.1));
#20147=CARTESIAN_POINT('',(12.0153882032022,-1.8,3.2));
#20148=CARTESIAN_POINT('Origin',(11.5,-1.9,3.2));
#20149=CARTESIAN_POINT('',(12.0153882032022,-1.8,3.1));
#20150=CARTESIAN_POINT('Origin',(8.5,1.9,3.8));
#20151=CARTESIAN_POINT('',(9.01538820320221,1.8,3.8));
#20152=CARTESIAN_POINT('',(7.98461179679779,1.8,3.8));
#20153=CARTESIAN_POINT('',(10.35,1.8,3.8));
#20154=CARTESIAN_POINT('Origin',(8.5,1.9,3.8));
#20155=CARTESIAN_POINT('Origin',(8.5,1.9,3.1));
#20156=CARTESIAN_POINT('',(9.01538820320221,1.8,3.2));
#20157=CARTESIAN_POINT('',(9.01538820320221,1.8,3.1));
#20158=CARTESIAN_POINT('',(7.98461179679779,1.8,3.2));
#20159=CARTESIAN_POINT('Origin',(8.5,1.9,3.2));
#20160=CARTESIAN_POINT('',(7.98461179679779,1.8,3.1));
#20161=CARTESIAN_POINT('Origin',(8.5,-1.9,3.8));
#20162=CARTESIAN_POINT('',(7.98461179679779,-1.8,3.8));
#20163=CARTESIAN_POINT('',(9.01538820320221,-1.8,3.8));
#20164=CARTESIAN_POINT('',(8.15,-1.8,3.8));
#20165=CARTESIAN_POINT('Origin',(8.5,-1.9,3.8));
#20166=CARTESIAN_POINT('Origin',(8.5,-1.9,3.1));
#20167=CARTESIAN_POINT('',(7.98461179679779,-1.8,3.2));
#20168=CARTESIAN_POINT('',(7.98461179679779,-1.8,3.1));
#20169=CARTESIAN_POINT('',(9.01538820320221,-1.8,3.2));
#20170=CARTESIAN_POINT('Origin',(8.5,-1.9,3.2));
#20171=CARTESIAN_POINT('',(9.01538820320221,-1.8,3.1));
#20172=CARTESIAN_POINT('Origin',(11.5,1.9,3.8));
#20173=CARTESIAN_POINT('',(12.0153882032022,1.8,3.8));
#20174=CARTESIAN_POINT('',(10.9846117967978,1.8,3.8));
#20175=CARTESIAN_POINT('',(11.85,1.8,3.8));
#20176=CARTESIAN_POINT('Origin',(11.5,1.9,3.8));
#20177=CARTESIAN_POINT('Origin',(11.5,1.9,3.1));
#20178=CARTESIAN_POINT('',(12.0153882032022,1.8,3.2));
#20179=CARTESIAN_POINT('',(12.0153882032022,1.8,3.1));
#20180=CARTESIAN_POINT('',(10.9846117967978,1.8,3.2));
#20181=CARTESIAN_POINT('Origin',(11.5,1.9,3.2));
#20182=CARTESIAN_POINT('',(10.9846117967978,1.8,3.1));
#20183=CARTESIAN_POINT('Origin',(7.8,-1.8,3.2));
#20184=CARTESIAN_POINT('',(13.4,-1.8,3.2));
#20185=CARTESIAN_POINT('',(6.6,-1.8,3.2));
#20186=CARTESIAN_POINT('',(13.4,-1.8,4.));
#20187=CARTESIAN_POINT('',(13.4,-1.8,3.2));
#20188=CARTESIAN_POINT('',(12.2,-1.8,4.));
#20189=CARTESIAN_POINT('',(13.4,-1.8,4.));
#20190=CARTESIAN_POINT('',(12.2,-1.8,9.2));
#20191=CARTESIAN_POINT('',(12.2,-1.8,3.2));
#20192=CARTESIAN_POINT('',(7.8,-1.8,9.2));
#20193=CARTESIAN_POINT('',(7.8,-1.8,9.2));
#20194=CARTESIAN_POINT('',(7.8,-1.8,4.));
#20195=CARTESIAN_POINT('',(7.8,-1.8,3.2));
#20196=CARTESIAN_POINT('',(6.6,-1.8,4.));
#20197=CARTESIAN_POINT('',(13.4,-1.8,4.));
#20198=CARTESIAN_POINT('',(6.6,-1.8,3.2));
#20199=CARTESIAN_POINT('',(6.6,-1.8,4.));
#20200=CARTESIAN_POINT('',(6.6,-1.8,3.2));
#20201=CARTESIAN_POINT('',(6.6,-1.8,3.2));
#20202=CARTESIAN_POINT('Origin',(12.2,1.8,3.2));
#20203=CARTESIAN_POINT('',(6.6,1.8,3.2));
#20204=CARTESIAN_POINT('',(6.6,1.8,3.2));
#20205=CARTESIAN_POINT('',(6.6,1.8,4.));
#20206=CARTESIAN_POINT('',(6.6,1.8,4.));
#20207=CARTESIAN_POINT('',(7.8,1.8,4.));
#20208=CARTESIAN_POINT('',(13.4,1.8,4.));
#20209=CARTESIAN_POINT('',(7.8,1.8,9.2));
#20210=CARTESIAN_POINT('',(7.8,1.8,3.2));
#20211=CARTESIAN_POINT('',(12.2,1.8,9.2));
#20212=CARTESIAN_POINT('',(12.2,1.8,9.2));
#20213=CARTESIAN_POINT('',(12.2,1.8,4.));
#20214=CARTESIAN_POINT('',(12.2,1.8,3.2));
#20215=CARTESIAN_POINT('',(13.4,1.8,4.));
#20216=CARTESIAN_POINT('',(13.4,1.8,4.));
#20217=CARTESIAN_POINT('',(13.4,1.8,3.2));
#20218=CARTESIAN_POINT('',(13.4,1.8,3.2));
#20219=CARTESIAN_POINT('',(6.6,1.8,3.2));
#20220=CARTESIAN_POINT('',(6.6,1.8,3.2));
#20221=CARTESIAN_POINT('Origin',(12.8,-1.,3.1));
#20222=CARTESIAN_POINT('',(12.575,-1.,3.2));
#20223=CARTESIAN_POINT('Origin',(12.8,-1.,3.2));
#20224=CARTESIAN_POINT('',(12.575,-1.,4.));
#20225=CARTESIAN_POINT('',(12.575,-1.,3.1));
#20226=CARTESIAN_POINT('Origin',(12.8,-1.,4.));
#20227=CARTESIAN_POINT('Origin',(7.2,1.,3.1));
#20228=CARTESIAN_POINT('',(6.975,1.,3.2));
#20229=CARTESIAN_POINT('Origin',(7.2,1.,3.2));
#20230=CARTESIAN_POINT('',(6.975,1.,4.));
#20231=CARTESIAN_POINT('',(6.975,1.,3.1));
#20232=CARTESIAN_POINT('Origin',(7.2,1.,4.));
#20233=CARTESIAN_POINT('Origin',(7.2,-1.,3.1));
#20234=CARTESIAN_POINT('',(6.975,-1.,3.2));
#20235=CARTESIAN_POINT('Origin',(7.2,-1.,3.2));
#20236=CARTESIAN_POINT('',(6.975,-1.,4.));
#20237=CARTESIAN_POINT('',(6.975,-1.,3.1));
#20238=CARTESIAN_POINT('Origin',(7.2,-1.,4.));
#20239=CARTESIAN_POINT('Origin',(12.8,1.,3.1));
#20240=CARTESIAN_POINT('',(12.575,1.,3.2));
#20241=CARTESIAN_POINT('Origin',(12.8,1.,3.2));
#20242=CARTESIAN_POINT('',(12.575,1.,4.));
#20243=CARTESIAN_POINT('',(12.575,1.,3.1));
#20244=CARTESIAN_POINT('Origin',(12.8,1.,4.));
#20245=CARTESIAN_POINT('Origin',(6.6,-1.8,4.));
#20246=CARTESIAN_POINT('',(12.2,-1.8,4.));
#20247=CARTESIAN_POINT('',(13.4,-1.8,4.));
#20248=CARTESIAN_POINT('Origin',(6.6,-1.8,4.));
#20249=CARTESIAN_POINT('',(7.8,0.,4.));
#20250=CARTESIAN_POINT('',(6.6,-1.8,4.));
#20251=CARTESIAN_POINT('Origin',(6.6,-1.8,3.2));
#20252=CARTESIAN_POINT('',(6.6,-1.8,3.2));
#20253=CARTESIAN_POINT('Origin',(13.4,-1.8,4.));
#20254=CARTESIAN_POINT('',(13.4,-1.8,3.2));
#20255=CARTESIAN_POINT('Origin',(12.2,-1.8,3.2));
#20256=CARTESIAN_POINT('',(12.2,-1.8,9.2));
#20257=CARTESIAN_POINT('Origin',(7.8,1.8,3.2));
#20258=CARTESIAN_POINT('',(7.8,1.8,9.2));
#20259=CARTESIAN_POINT('Origin',(10.,0.,9.2));
#20260=CARTESIAN_POINT('Origin',(10.,0.,3.2));
#23482=UNCERTAINTY_MEASURE_WITH_UNIT(LENGTH_MEASURE(0.001),#23588,
'DISTANCE_ACCURACY_VALUE',
'Maximum model space distance between geometric entities at asserted c
onnectivities');
#23522=UNCERTAINTY_MEASURE_WITH_UNIT(LENGTH_MEASURE(0.001),#23588,
'DISTANCE_ACCURACY_VALUE',
'Maximum model space distance between geometric entities at asserted c
onnectivities');
#23547=(
GEOMETRIC_REPRESENTATION_CONTEXT(3)
GLOBAL_UNCERTAINTY_ASSIGNED_CONTEXT((#23482))
GLOBAL_UNIT_ASSIGNED_CONTEXT((#23588,#23590,#23591))
REPRESENTATION_CONTEXT('','3D')
);
#23587=(
GEOMETRIC_REPRESENTATION_CONTEXT(3)
GLOBAL_UNCERTAINTY_ASSIGNED_CONTEXT((#23522))
GLOBAL_UNIT_ASSIGNED_CONTEXT((#23588,#23590,#23591))
REPRESENTATION_CONTEXT('','3D')
);
#23588=(
LENGTH_UNIT()
NAMED_UNIT(*)
SI_UNIT(.CENTI.,.METRE.)
);
#23590=(
NAMED_UNIT(*)
PLANE_ANGLE_UNIT()
SI_UNIT($,.RADIAN.)
);
#23591=(
NAMED_UNIT(*)
SI_UNIT($,.STERADIAN.)
SOLID_ANGLE_UNIT()
);
#23616=SHAPE_DEFINITION_REPRESENTATION(#23685,#23849);
#23685=PRODUCT_DEFINITION_SHAPE('',$,#23914);
#23849=SHAPE_REPRESENTATION('',(#13393),#23547);
#23889=PRODUCT_DEFINITION_CONTEXT('part definition',#24083,'design');
#23914=PRODUCT_DEFINITION('Sliding bearing block',
'Sliding bearing block',#23978,#23889);
#23978=PRODUCT_DEFINITION_FORMATION('',$,#24109);
#24083=APPLICATION_CONTEXT(
'Core Data for Automotive Mechanical Design Process');
#24084=PRODUCT_CONTEXT('part definition',#24083,'mechanical');
#24109=PRODUCT('Sliding bearing block','Sliding bearing block',
'Sliding bearing block',(#24084));
#24205=COLOUR_RGB('Grey',0.48,0.52,0.57);
#24206=FILL_AREA_STYLE_COLOUR('',#24205);
#24207=FILL_AREA_STYLE('',(#24206));
#24208=SURFACE_STYLE_FILL_AREA(#24207);
#24209=SURFACE_SIDE_STYLE('',(#24208));
#24210=SURFACE_STYLE_USAGE(.BOTH.,#24209);
#24211=PRESENTATION_STYLE_ASSIGNMENT((#24210));
ENDSEC;
END-ISO-10303-21;
